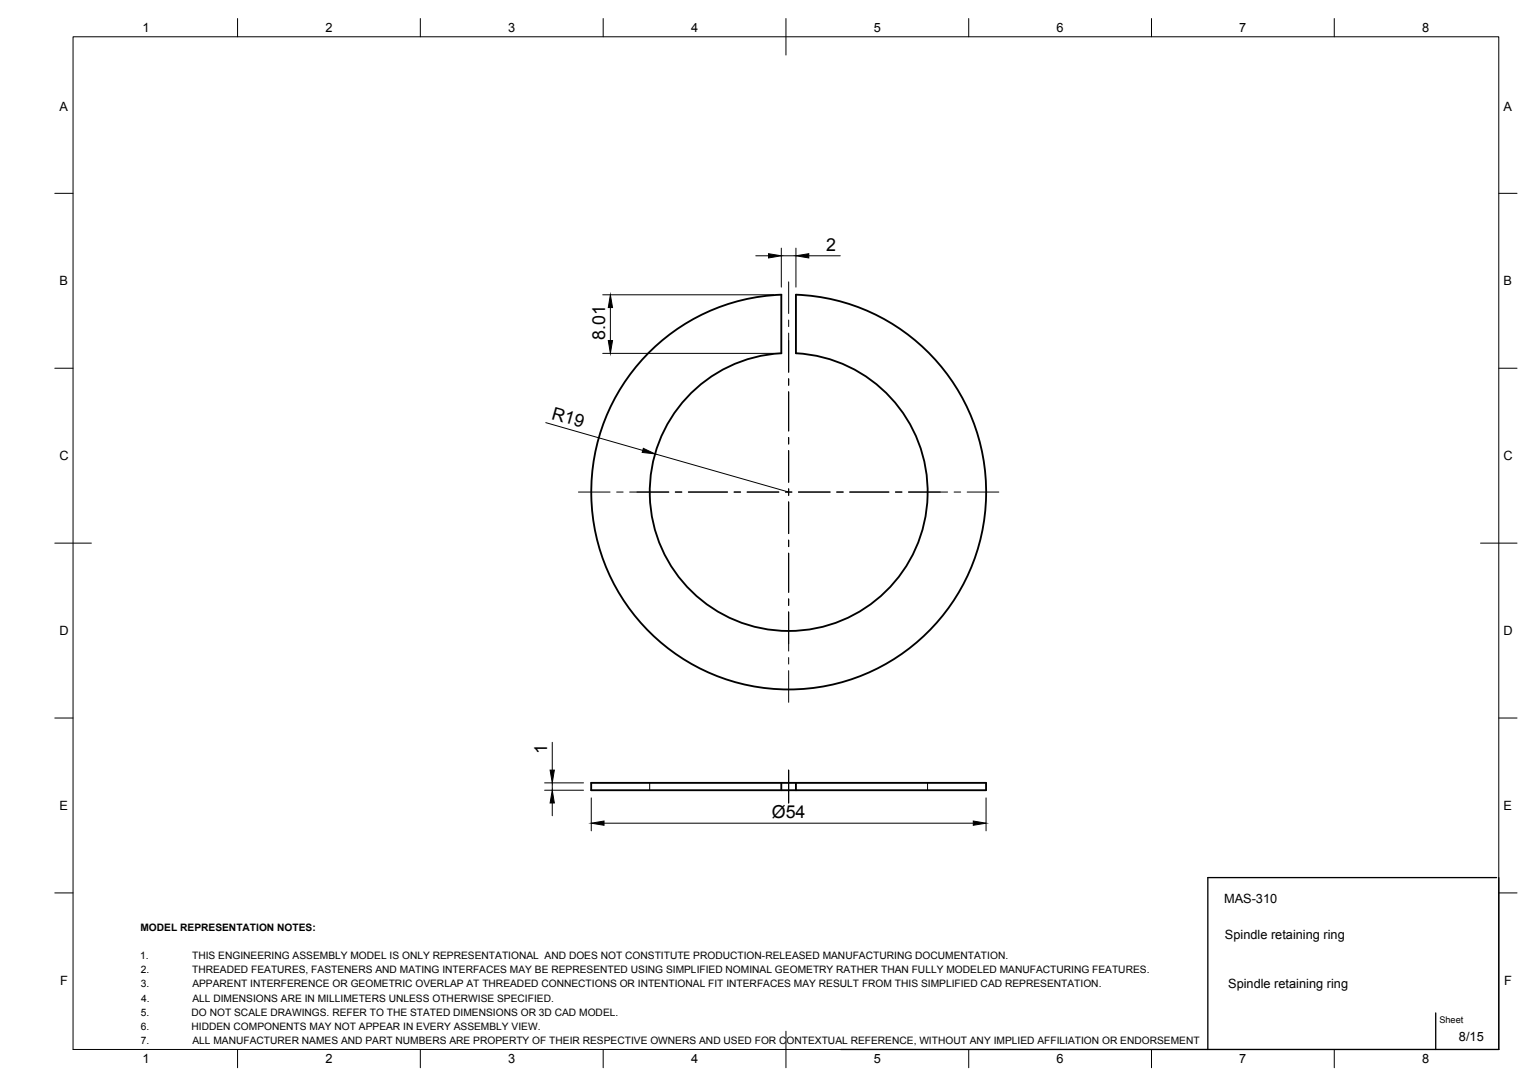
ISO-10303-21;
HEADER;
/* Generated by software containing ST-Developer
 * from STEP Tools, Inc. (www.steptools.com) 
 */

FILE_DESCRIPTION(
/* description */ ('Independent30mm screw-fed quill/spindle unit with16mm straight tool s
ocket, radial set screw, native reusable open ball bearings, retained 
inner/outer race stacks, keyed quill guide and M12x1.75 fine feed. Ext
ernal moving drive and tool not included. Ideal cage orbital links; in
dividual ball spin, force and preload not simulated. No drilling capac
ity, runout, speed, torque, load, life or machine safety rating.'),
/* implementation_level */ '2;1');

FILE_NAME(
/* name */ 'Spindle retaining ring.step',
/* time_stamp */ '2026-11-08T18:59:42-08:00',
/* author */ (''),
/* organization */ (''),
/* preprocessor_version */ 'ST-DEVELOPER v20.2',
/* originating_system */ 'Autodesk Translation Framework v15.17.0.0',
/* authorisation */ '');

FILE_SCHEMA (('AUTOMOTIVE_DESIGN { 1 0 10303 214 3 1 1 }'));
ENDSEC;

DATA;
#10=MECHANICAL_DESIGN_GEOMETRIC_PRESENTATION_REPRESENTATION('',(#1597),#63898);
#1561=SHAPE_REPRESENTATION_RELATIONSHIP('SRR','None',#64000,#1579);
#1579=ADVANCED_BREP_SHAPE_REPRESENTATION('',(#1615),#63885);
#1597=STYLED_ITEM('',(#64099),#1615);
#1615=MANIFOLD_SOLID_BREP('Body1',#15483);
#2110=CYLINDRICAL_SURFACE('',#16292,19.);
#2111=CYLINDRICAL_SURFACE('',#16294,27.);
#2507=CIRCLE('',#16290,27.);
#2508=CIRCLE('',#16291,19.);
#2509=CIRCLE('',#16293,19.);
#2510=CIRCLE('',#16295,27.);
#3138=FACE_OUTER_BOUND('',#4021,.T.);
#3139=FACE_OUTER_BOUND('',#4022,.T.);
#3140=FACE_OUTER_BOUND('',#4023,.T.);
#3141=FACE_OUTER_BOUND('',#4024,.T.);
#3142=FACE_OUTER_BOUND('',#4025,.T.);
#3143=FACE_OUTER_BOUND('',#4026,.T.);
#4021=EDGE_LOOP('',(#12520,#12521,#12522,#12523));
#4022=EDGE_LOOP('',(#12524,#12525,#12526,#12527));
#4023=EDGE_LOOP('',(#12528,#12529,#12530,#12531));
#4024=EDGE_LOOP('',(#12532,#12533,#12534,#12535));
#4025=EDGE_LOOP('',(#12536,#12537,#12538,#12539));
#4026=EDGE_LOOP('',(#12540,#12541,#12542,#12543));
#4860=LINE('',#46789,#5623);
#4861=LINE('',#46791,#5624);
#4862=LINE('',#46793,#5625);
#4863=LINE('',#46794,#5626);
#4864=LINE('',#46798,#5627);
#4865=LINE('',#46800,#5628);
#4866=LINE('',#46802,#5629);
#4867=LINE('',#46803,#5630);
#5623=VECTOR('',#18482,10.);
#5624=VECTOR('',#18483,10.);
#5625=VECTOR('',#18484,10.);
#5626=VECTOR('',#18485,10.);
#5627=VECTOR('',#18488,10.);
#5628=VECTOR('',#18489,10.);
#5629=VECTOR('',#18490,10.);
#5630=VECTOR('',#18491,10.);
#6840=VERTEX_POINT('',#46787);
#6841=VERTEX_POINT('',#46788);
#6842=VERTEX_POINT('',#46790);
#6843=VERTEX_POINT('',#46792);
#6844=VERTEX_POINT('',#46796);
#6845=VERTEX_POINT('',#46797);
#6846=VERTEX_POINT('',#46799);
#6847=VERTEX_POINT('',#46801);
#8849=EDGE_CURVE('',#6840,#6841,#4860,.T.);
#8850=EDGE_CURVE('',#6842,#6840,#4861,.T.);
#8851=EDGE_CURVE('',#6843,#6842,#4862,.T.);
#8852=EDGE_CURVE('',#6841,#6843,#4863,.T.);
#8853=EDGE_CURVE('',#6844,#6845,#4864,.T.);
#8854=EDGE_CURVE('',#6846,#6844,#4865,.T.);
#8855=EDGE_CURVE('',#6847,#6846,#4866,.T.);
#8856=EDGE_CURVE('',#6845,#6847,#4867,.T.);
#8857=EDGE_CURVE('',#6842,#6847,#2507,.T.);
#8858=EDGE_CURVE('',#6845,#6840,#2508,.T.);
#8859=EDGE_CURVE('',#6844,#6841,#2509,.T.);
#8860=EDGE_CURVE('',#6843,#6846,#2510,.T.);
#12520=ORIENTED_EDGE('',*,*,#8849,.F.);
#12521=ORIENTED_EDGE('',*,*,#8850,.F.);
#12522=ORIENTED_EDGE('',*,*,#8851,.F.);
#12523=ORIENTED_EDGE('',*,*,#8852,.F.);
#12524=ORIENTED_EDGE('',*,*,#8853,.F.);
#12525=ORIENTED_EDGE('',*,*,#8854,.F.);
#12526=ORIENTED_EDGE('',*,*,#8855,.F.);
#12527=ORIENTED_EDGE('',*,*,#8856,.F.);
#12528=ORIENTED_EDGE('',*,*,#8856,.T.);
#12529=ORIENTED_EDGE('',*,*,#8857,.F.);
#12530=ORIENTED_EDGE('',*,*,#8850,.T.);
#12531=ORIENTED_EDGE('',*,*,#8858,.F.);
#12532=ORIENTED_EDGE('',*,*,#8853,.T.);
#12533=ORIENTED_EDGE('',*,*,#8858,.T.);
#12534=ORIENTED_EDGE('',*,*,#8849,.T.);
#12535=ORIENTED_EDGE('',*,*,#8859,.F.);
#12536=ORIENTED_EDGE('',*,*,#8855,.T.);
#12537=ORIENTED_EDGE('',*,*,#8860,.F.);
#12538=ORIENTED_EDGE('',*,*,#8851,.T.);
#12539=ORIENTED_EDGE('',*,*,#8857,.T.);
#12540=ORIENTED_EDGE('',*,*,#8854,.T.);
#12541=ORIENTED_EDGE('',*,*,#8859,.T.);
#12542=ORIENTED_EDGE('',*,*,#8852,.T.);
#12543=ORIENTED_EDGE('',*,*,#8860,.T.);
#14573=PLANE('',#16287);
#14574=PLANE('',#16288);
#14575=PLANE('',#16289);
#14576=PLANE('',#16296);
#15118=ADVANCED_FACE('',(#3138),#14573,.F.);
#15119=ADVANCED_FACE('',(#3139),#14574,.F.);
#15120=ADVANCED_FACE('',(#3140),#14575,.F.);
#15121=ADVANCED_FACE('',(#3141),#2110,.F.);
#15122=ADVANCED_FACE('',(#3142),#2111,.T.);
#15123=ADVANCED_FACE('',(#3143),#14576,.T.);
#15483=CLOSED_SHELL('',(#15118,#15119,#15120,#15121,#15122,#15123));
#16286=AXIS2_PLACEMENT_3D('',#46785,#18478,#18479);
#16287=AXIS2_PLACEMENT_3D('',#46786,#18480,#18481);
#16288=AXIS2_PLACEMENT_3D('',#46795,#18486,#18487);
#16289=AXIS2_PLACEMENT_3D('',#46804,#18492,#18493);
#16290=AXIS2_PLACEMENT_3D('',#46805,#18494,#18495);
#16291=AXIS2_PLACEMENT_3D('',#46806,#18496,#18497);
#16292=AXIS2_PLACEMENT_3D('',#46807,#18498,#18499);
#16293=AXIS2_PLACEMENT_3D('',#46808,#18500,#18501);
#16294=AXIS2_PLACEMENT_3D('',#46809,#18502,#18503);
#16295=AXIS2_PLACEMENT_3D('',#46810,#18504,#18505);
#16296=AXIS2_PLACEMENT_3D('',#46811,#18506,#18507);
#18478=DIRECTION('axis',(0.,0.,1.));
#18479=DIRECTION('refdir',(1.,0.,0.));
#18480=DIRECTION('center_axis',(-1.,0.,0.));
#18481=DIRECTION('ref_axis',(0.,1.,0.));
#18482=DIRECTION('',(0.,0.,1.));
#18483=DIRECTION('',(0.,-1.,0.));
#18484=DIRECTION('',(0.,0.,-1.));
#18485=DIRECTION('',(0.,1.,0.));
#18486=DIRECTION('center_axis',(1.,0.,0.));
#18487=DIRECTION('ref_axis',(0.,-1.,0.));
#18488=DIRECTION('',(0.,0.,-1.));
#18489=DIRECTION('',(0.,-1.,0.));
#18490=DIRECTION('',(0.,0.,1.));
#18491=DIRECTION('',(0.,1.,0.));
#18492=DIRECTION('center_axis',(0.,0.,1.));
#18493=DIRECTION('ref_axis',(1.,0.,0.));
#18494=DIRECTION('center_axis',(0.,0.,1.));
#18495=DIRECTION('ref_axis',(1.,0.,0.));
#18496=DIRECTION('center_axis',(0.,0.,-1.));
#18497=DIRECTION('ref_axis',(1.,0.,0.));
#18498=DIRECTION('center_axis',(0.,0.,1.));
#18499=DIRECTION('ref_axis',(6.12323399573677E-17,-1.,0.));
#18500=DIRECTION('center_axis',(0.,0.,-1.));
#18501=DIRECTION('ref_axis',(1.,0.,0.));
#18502=DIRECTION('center_axis',(0.,0.,1.));
#18503=DIRECTION('ref_axis',(6.12323399573677E-17,-1.,0.));
#18504=DIRECTION('center_axis',(0.,0.,1.));
#18505=DIRECTION('ref_axis',(1.,0.,0.));
#18506=DIRECTION('center_axis',(0.,0.,1.));
#18507=DIRECTION('ref_axis',(1.,0.,0.));
#46785=CARTESIAN_POINT('',(0.,0.,0.));
#46786=CARTESIAN_POINT('Origin',(-1.,0.,1.));
#46787=CARTESIAN_POINT('',(-1.,18.9736659610103,0.));
#46788=CARTESIAN_POINT('',(-1.,18.9736659610103,1.));
#46789=CARTESIAN_POINT('',(-1.,18.9736659610103,0.));
#46790=CARTESIAN_POINT('',(-1.,26.9814751264641,0.));
#46791=CARTESIAN_POINT('',(-1.,0.,0.));
#46792=CARTESIAN_POINT('',(-1.,26.9814751264641,1.));
#46793=CARTESIAN_POINT('',(-1.,26.9814751264641,0.));
#46794=CARTESIAN_POINT('',(-1.,0.,1.));
#46795=CARTESIAN_POINT('Origin',(1.,54.,1.));
#46796=CARTESIAN_POINT('',(1.,18.9736659610103,1.));
#46797=CARTESIAN_POINT('',(1.,18.9736659610103,0.));
#46798=CARTESIAN_POINT('',(1.,18.9736659610103,0.));
#46799=CARTESIAN_POINT('',(1.,26.9814751264641,1.));
#46800=CARTESIAN_POINT('',(1.,27.,1.));
#46801=CARTESIAN_POINT('',(1.,26.9814751264641,0.));
#46802=CARTESIAN_POINT('',(1.,26.9814751264641,0.));
#46803=CARTESIAN_POINT('',(1.,27.,0.));
#46804=CARTESIAN_POINT('Origin',(0.,0.,0.));
#46805=CARTESIAN_POINT('Origin',(0.,0.,0.));
#46806=CARTESIAN_POINT('Origin',(0.,0.,0.));
#46807=CARTESIAN_POINT('Origin',(0.,0.,0.));
#46808=CARTESIAN_POINT('Origin',(0.,0.,1.));
#46809=CARTESIAN_POINT('Origin',(0.,0.,0.));
#46810=CARTESIAN_POINT('Origin',(0.,0.,1.));
#46811=CARTESIAN_POINT('Origin',(0.,0.,1.));
#63865=UNCERTAINTY_MEASURE_WITH_UNIT(LENGTH_MEASURE(0.01),#63899,
'DISTANCE_ACCURACY_VALUE',
'Maximum model space distance between geometric entities at asserted c
onnectivities');
#63878=UNCERTAINTY_MEASURE_WITH_UNIT(LENGTH_MEASURE(0.01),#63899,
'DISTANCE_ACCURACY_VALUE',
'Maximum model space distance between geometric entities at asserted c
onnectivities');
#63885=(
GEOMETRIC_REPRESENTATION_CONTEXT(3)
GLOBAL_UNCERTAINTY_ASSIGNED_CONTEXT((#63865))
GLOBAL_UNIT_ASSIGNED_CONTEXT((#63899,#63901,#63902))
REPRESENTATION_CONTEXT('','3D')
);
#63898=(
GEOMETRIC_REPRESENTATION_CONTEXT(3)
GLOBAL_UNCERTAINTY_ASSIGNED_CONTEXT((#63878))
GLOBAL_UNIT_ASSIGNED_CONTEXT((#63899,#63901,#63902))
REPRESENTATION_CONTEXT('','3D')
);
#63899=(
LENGTH_UNIT()
NAMED_UNIT(*)
SI_UNIT(.MILLI.,.METRE.)
);
#63901=(
NAMED_UNIT(*)
PLANE_ANGLE_UNIT()
SI_UNIT($,.RADIAN.)
);
#63902=(
NAMED_UNIT(*)
SI_UNIT($,.STERADIAN.)
SOLID_ANGLE_UNIT()
);
#63909=SHAPE_DEFINITION_REPRESENTATION(#63928,#64000);
#63928=PRODUCT_DEFINITION_SHAPE('',$,#64020);
#64000=SHAPE_REPRESENTATION('',(#16286),#63885);
#64013=PRODUCT_DEFINITION_CONTEXT('part definition',#64072,'design');
#64020=PRODUCT_DEFINITION('Spindle retaining ring',
'Spindle retaining ring',#64039,#64013);
#64039=PRODUCT_DEFINITION_FORMATION('',$,#64080);
#64072=APPLICATION_CONTEXT(
'Core Data for Automotive Mechanical Design Process');
#64073=PRODUCT_CONTEXT('part definition',#64072,'mechanical');
#64080=PRODUCT('Spindle retaining ring','Spindle retaining ring',$,(#64073));
#64099=PRESENTATION_STYLE_ASSIGNMENT((#64112));
#64112=SURFACE_STYLE_USAGE(.BOTH.,#64125);
#64125=SURFACE_SIDE_STYLE('',(#64138));
#64138=SURFACE_STYLE_FILL_AREA(#64151);
#64151=FILL_AREA_STYLE('Dark gray',(#64164));
#64164=FILL_AREA_STYLE_COLOUR('Dark gray',#64177);
#64177=COLOUR_RGB('Dark gray',0.250980392156863,0.282352941176471,0.32156862745098);
ENDSEC;
END-ISO-10303-21;
